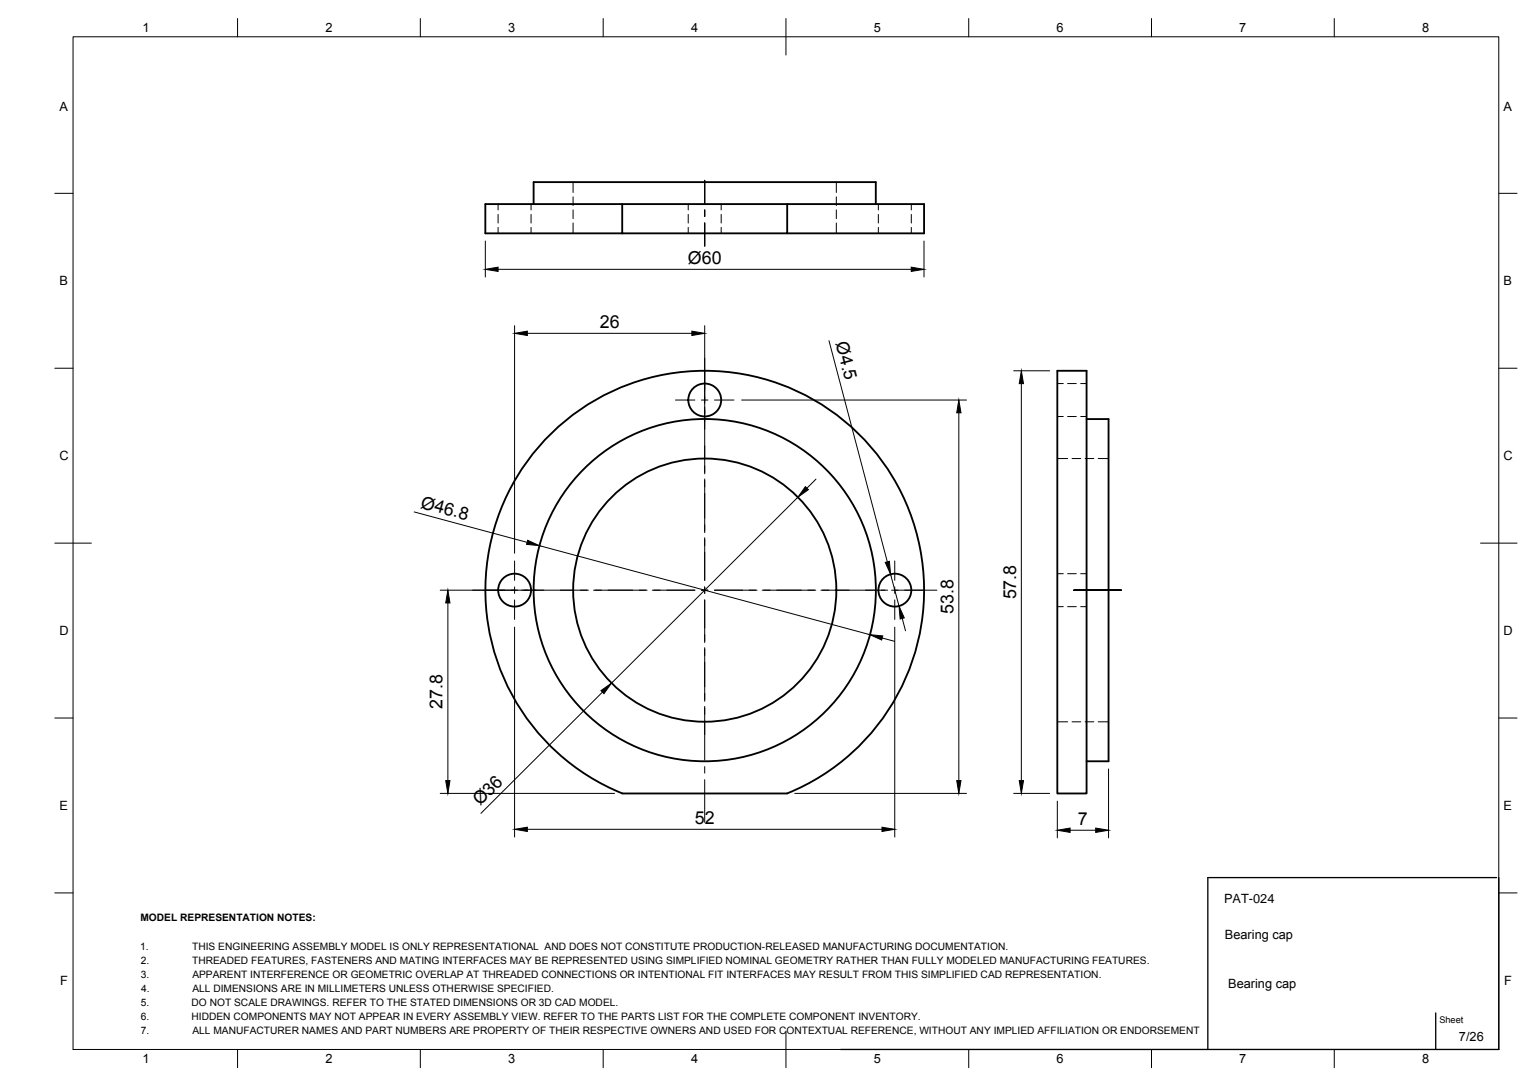
ISO-10303-21;
HEADER;
/* Generated by software containing ST-Developer
 * from STEP Tools, Inc. (www.steptools.com) 
 */

FILE_DESCRIPTION(
/* description */ ('Compact handwheel screw vise'),
/* implementation_level */ '2;1');

FILE_NAME(
/* name */ 'Bearing cap.step',
/* time_stamp */ '2026-10-29T16:08:22-07:00',
/* author */ (''),
/* organization */ (''),
/* preprocessor_version */ 'ST-DEVELOPER v20.2',
/* originating_system */ 'Autodesk Translation Framework v15.17.0.0',
/* authorisation */ '');

FILE_SCHEMA (('AUTOMOTIVE_DESIGN { 1 0 10303 214 3 1 1 }'));
ENDSEC;

DATA;
#10=MECHANICAL_DESIGN_GEOMETRIC_PRESENTATION_REPRESENTATION('',(#648),#25074);
#592=SHAPE_REPRESENTATION_RELATIONSHIP('SRR','None',#25200,#620);
#620=ADVANCED_BREP_SHAPE_REPRESENTATION('',(#684),#25047);
#648=STYLED_ITEM('',(#25439),#684);
#684=MANIFOLD_SOLID_BREP('Body1',#8056);
#744=FACE_BOUND('',#1574,.T.);
#745=FACE_BOUND('',#1575,.T.);
#746=FACE_BOUND('',#1576,.T.);
#747=FACE_BOUND('',#1577,.T.);
#748=FACE_BOUND('',#1581,.T.);
#749=FACE_BOUND('',#1584,.T.);
#750=FACE_BOUND('',#1585,.T.);
#751=FACE_BOUND('',#1586,.T.);
#752=FACE_BOUND('',#1587,.T.);
#856=PLANE('',#8514);
#857=PLANE('',#8515);
#858=PLANE('',#8522);
#859=PLANE('',#8526);
#1067=FACE_OUTER_BOUND('',#1569,.T.);
#1068=FACE_OUTER_BOUND('',#1570,.T.);
#1069=FACE_OUTER_BOUND('',#1571,.T.);
#1070=FACE_OUTER_BOUND('',#1572,.T.);
#1071=FACE_OUTER_BOUND('',#1573,.T.);
#1072=FACE_OUTER_BOUND('',#1578,.T.);
#1073=FACE_OUTER_BOUND('',#1579,.T.);
#1074=FACE_OUTER_BOUND('',#1580,.T.);
#1075=FACE_OUTER_BOUND('',#1582,.T.);
#1076=FACE_OUTER_BOUND('',#1583,.T.);
#1569=EDGE_LOOP('',(#5381,#5382,#5383,#5384));
#1570=EDGE_LOOP('',(#5385,#5386,#5387,#5388));
#1571=EDGE_LOOP('',(#5389,#5390,#5391,#5392));
#1572=EDGE_LOOP('',(#5393,#5394,#5395,#5396));
#1573=EDGE_LOOP('',(#5397,#5398));
#1574=EDGE_LOOP('',(#5399));
#1575=EDGE_LOOP('',(#5400));
#1576=EDGE_LOOP('',(#5401));
#1577=EDGE_LOOP('',(#5402));
#1578=EDGE_LOOP('',(#5403,#5404,#5405,#5406));
#1579=EDGE_LOOP('',(#5407,#5408,#5409,#5410));
#1580=EDGE_LOOP('',(#5411));
#1581=EDGE_LOOP('',(#5412));
#1582=EDGE_LOOP('',(#5413,#5414,#5415,#5416));
#1583=EDGE_LOOP('',(#5417,#5418));
#1584=EDGE_LOOP('',(#5419));
#1585=EDGE_LOOP('',(#5420));
#1586=EDGE_LOOP('',(#5421));
#1587=EDGE_LOOP('',(#5422));
#2131=LINE('',#11569,#2639);
#2132=LINE('',#11575,#2640);
#2133=LINE('',#11581,#2641);
#2134=LINE('',#11586,#2642);
#2135=LINE('',#11588,#2643);
#2136=LINE('',#11590,#2644);
#2137=LINE('',#11591,#2645);
#2138=LINE('',#11600,#2646);
#2139=LINE('',#11608,#2647);
#2639=VECTOR('',#9485,0.225);
#2640=VECTOR('',#9492,0.225);
#2641=VECTOR('',#9499,0.225);
#2642=VECTOR('',#9504,1.);
#2643=VECTOR('',#9505,1.);
#2644=VECTOR('',#9506,1.);
#2645=VECTOR('',#9507,1.);
#2646=VECTOR('',#9520,2.34);
#2647=VECTOR('',#9531,1.8);
#3120=CIRCLE('',#8506,0.225);
#3121=CIRCLE('',#8507,0.225);
#3122=CIRCLE('',#8509,0.225);
#3123=CIRCLE('',#8510,0.225);
#3124=CIRCLE('',#8512,0.225);
#3125=CIRCLE('',#8513,0.225);
#3126=CIRCLE('',#8516,3.);
#3127=CIRCLE('',#8517,2.34);
#3128=CIRCLE('',#8519,3.);
#3129=CIRCLE('',#8521,2.34);
#3130=CIRCLE('',#8523,1.8);
#3131=CIRCLE('',#8525,1.8);
#3407=VERTEX_POINT('',#11566);
#3408=VERTEX_POINT('',#11568);
#3409=VERTEX_POINT('',#11572);
#3410=VERTEX_POINT('',#11574);
#3411=VERTEX_POINT('',#11578);
#3412=VERTEX_POINT('',#11580);
#3413=VERTEX_POINT('',#11584);
#3414=VERTEX_POINT('',#11585);
#3415=VERTEX_POINT('',#11587);
#3416=VERTEX_POINT('',#11589);
#3417=VERTEX_POINT('',#11594);
#3418=VERTEX_POINT('',#11599);
#3419=VERTEX_POINT('',#11603);
#3420=VERTEX_POINT('',#11606);
#4177=EDGE_CURVE('',#3407,#3407,#3120,.T.);
#4178=EDGE_CURVE('',#3407,#3408,#2131,.T.);
#4179=EDGE_CURVE('',#3408,#3408,#3121,.T.);
#4180=EDGE_CURVE('',#3409,#3409,#3122,.T.);
#4181=EDGE_CURVE('',#3409,#3410,#2132,.T.);
#4182=EDGE_CURVE('',#3410,#3410,#3123,.T.);
#4183=EDGE_CURVE('',#3411,#3411,#3124,.T.);
#4184=EDGE_CURVE('',#3411,#3412,#2133,.T.);
#4185=EDGE_CURVE('',#3412,#3412,#3125,.T.);
#4186=EDGE_CURVE('',#3413,#3414,#2134,.T.);
#4187=EDGE_CURVE('',#3415,#3413,#2135,.T.);
#4188=EDGE_CURVE('',#3416,#3415,#2136,.T.);
#4189=EDGE_CURVE('',#3414,#3416,#2137,.T.);
#4190=EDGE_CURVE('',#3415,#3413,#3126,.T.);
#4191=EDGE_CURVE('',#3417,#3417,#3127,.T.);
#4192=EDGE_CURVE('',#3416,#3414,#3128,.T.);
#4193=EDGE_CURVE('',#3417,#3418,#2138,.T.);
#4194=EDGE_CURVE('',#3418,#3418,#3129,.T.);
#4195=EDGE_CURVE('',#3419,#3419,#3130,.T.);
#4196=EDGE_CURVE('',#3420,#3420,#3131,.T.);
#4197=EDGE_CURVE('',#3420,#3419,#2139,.T.);
#5381=ORIENTED_EDGE('',*,*,#4177,.F.);
#5382=ORIENTED_EDGE('',*,*,#4178,.T.);
#5383=ORIENTED_EDGE('',*,*,#4179,.F.);
#5384=ORIENTED_EDGE('',*,*,#4178,.F.);
#5385=ORIENTED_EDGE('',*,*,#4180,.F.);
#5386=ORIENTED_EDGE('',*,*,#4181,.T.);
#5387=ORIENTED_EDGE('',*,*,#4182,.F.);
#5388=ORIENTED_EDGE('',*,*,#4181,.F.);
#5389=ORIENTED_EDGE('',*,*,#4183,.F.);
#5390=ORIENTED_EDGE('',*,*,#4184,.T.);
#5391=ORIENTED_EDGE('',*,*,#4185,.F.);
#5392=ORIENTED_EDGE('',*,*,#4184,.F.);
#5393=ORIENTED_EDGE('',*,*,#4186,.F.);
#5394=ORIENTED_EDGE('',*,*,#4187,.F.);
#5395=ORIENTED_EDGE('',*,*,#4188,.F.);
#5396=ORIENTED_EDGE('',*,*,#4189,.F.);
#5397=ORIENTED_EDGE('',*,*,#4187,.T.);
#5398=ORIENTED_EDGE('',*,*,#4190,.F.);
#5399=ORIENTED_EDGE('',*,*,#4177,.T.);
#5400=ORIENTED_EDGE('',*,*,#4180,.T.);
#5401=ORIENTED_EDGE('',*,*,#4183,.T.);
#5402=ORIENTED_EDGE('',*,*,#4191,.T.);
#5403=ORIENTED_EDGE('',*,*,#4188,.T.);
#5404=ORIENTED_EDGE('',*,*,#4190,.T.);
#5405=ORIENTED_EDGE('',*,*,#4186,.T.);
#5406=ORIENTED_EDGE('',*,*,#4192,.F.);
#5407=ORIENTED_EDGE('',*,*,#4191,.F.);
#5408=ORIENTED_EDGE('',*,*,#4193,.T.);
#5409=ORIENTED_EDGE('',*,*,#4194,.T.);
#5410=ORIENTED_EDGE('',*,*,#4193,.F.);
#5411=ORIENTED_EDGE('',*,*,#4194,.F.);
#5412=ORIENTED_EDGE('',*,*,#4195,.F.);
#5413=ORIENTED_EDGE('',*,*,#4196,.F.);
#5414=ORIENTED_EDGE('',*,*,#4197,.T.);
#5415=ORIENTED_EDGE('',*,*,#4195,.T.);
#5416=ORIENTED_EDGE('',*,*,#4197,.F.);
#5417=ORIENTED_EDGE('',*,*,#4189,.T.);
#5418=ORIENTED_EDGE('',*,*,#4192,.T.);
#5419=ORIENTED_EDGE('',*,*,#4179,.T.);
#5420=ORIENTED_EDGE('',*,*,#4182,.T.);
#5421=ORIENTED_EDGE('',*,*,#4185,.T.);
#5422=ORIENTED_EDGE('',*,*,#4196,.T.);
#7366=CYLINDRICAL_SURFACE('',#8505,0.225);
#7367=CYLINDRICAL_SURFACE('',#8508,0.225);
#7368=CYLINDRICAL_SURFACE('',#8511,0.225);
#7369=CYLINDRICAL_SURFACE('',#8518,3.);
#7370=CYLINDRICAL_SURFACE('',#8520,2.34);
#7371=CYLINDRICAL_SURFACE('',#8524,1.8);
#7637=ADVANCED_FACE('',(#1067),#7366,.F.);
#7638=ADVANCED_FACE('',(#1068),#7367,.F.);
#7639=ADVANCED_FACE('',(#1069),#7368,.F.);
#7640=ADVANCED_FACE('',(#1070),#856,.F.);
#7641=ADVANCED_FACE('',(#1071,#744,#745,#746,#747),#857,.F.);
#7642=ADVANCED_FACE('',(#1072),#7369,.T.);
#7643=ADVANCED_FACE('',(#1073),#7370,.T.);
#7644=ADVANCED_FACE('',(#1074,#748),#858,.F.);
#7645=ADVANCED_FACE('',(#1075),#7371,.F.);
#7646=ADVANCED_FACE('',(#1076,#749,#750,#751,#752),#859,.T.);
#8056=CLOSED_SHELL('',(#7637,#7638,#7639,#7640,#7641,#7642,#7643,#7644,
#7645,#7646));
#8504=AXIS2_PLACEMENT_3D('',#11564,#9479,#9480);
#8505=AXIS2_PLACEMENT_3D('',#11565,#9481,#9482);
#8506=AXIS2_PLACEMENT_3D('',#11567,#9483,#9484);
#8507=AXIS2_PLACEMENT_3D('',#11570,#9486,#9487);
#8508=AXIS2_PLACEMENT_3D('',#11571,#9488,#9489);
#8509=AXIS2_PLACEMENT_3D('',#11573,#9490,#9491);
#8510=AXIS2_PLACEMENT_3D('',#11576,#9493,#9494);
#8511=AXIS2_PLACEMENT_3D('',#11577,#9495,#9496);
#8512=AXIS2_PLACEMENT_3D('',#11579,#9497,#9498);
#8513=AXIS2_PLACEMENT_3D('',#11582,#9500,#9501);
#8514=AXIS2_PLACEMENT_3D('',#11583,#9502,#9503);
#8515=AXIS2_PLACEMENT_3D('',#11592,#9508,#9509);
#8516=AXIS2_PLACEMENT_3D('',#11593,#9510,#9511);
#8517=AXIS2_PLACEMENT_3D('',#11595,#9512,#9513);
#8518=AXIS2_PLACEMENT_3D('',#11596,#9514,#9515);
#8519=AXIS2_PLACEMENT_3D('',#11597,#9516,#9517);
#8520=AXIS2_PLACEMENT_3D('',#11598,#9518,#9519);
#8521=AXIS2_PLACEMENT_3D('',#11601,#9521,#9522);
#8522=AXIS2_PLACEMENT_3D('',#11602,#9523,#9524);
#8523=AXIS2_PLACEMENT_3D('',#11604,#9525,#9526);
#8524=AXIS2_PLACEMENT_3D('',#11605,#9527,#9528);
#8525=AXIS2_PLACEMENT_3D('',#11607,#9529,#9530);
#8526=AXIS2_PLACEMENT_3D('',#11609,#9532,#9533);
#9479=DIRECTION('axis',(0.,0.,1.));
#9480=DIRECTION('refdir',(1.,0.,0.));
#9481=DIRECTION('center_axis',(1.,0.,0.));
#9482=DIRECTION('ref_axis',(0.,0.,-1.));
#9483=DIRECTION('center_axis',(1.,0.,0.));
#9484=DIRECTION('ref_axis',(0.,0.,-1.));
#9485=DIRECTION('',(1.,0.,0.));
#9486=DIRECTION('center_axis',(-1.,0.,0.));
#9487=DIRECTION('ref_axis',(0.,0.,-1.));
#9488=DIRECTION('center_axis',(1.,0.,0.));
#9489=DIRECTION('ref_axis',(0.,0.,-1.));
#9490=DIRECTION('center_axis',(1.,0.,0.));
#9491=DIRECTION('ref_axis',(0.,0.,-1.));
#9492=DIRECTION('',(1.,0.,0.));
#9493=DIRECTION('center_axis',(-1.,0.,0.));
#9494=DIRECTION('ref_axis',(0.,0.,-1.));
#9495=DIRECTION('center_axis',(1.,0.,0.));
#9496=DIRECTION('ref_axis',(0.,0.,-1.));
#9497=DIRECTION('center_axis',(1.,0.,0.));
#9498=DIRECTION('ref_axis',(0.,0.,-1.));
#9499=DIRECTION('',(1.,0.,0.));
#9500=DIRECTION('center_axis',(-1.,0.,0.));
#9501=DIRECTION('ref_axis',(0.,0.,-1.));
#9502=DIRECTION('center_axis',(0.,0.,1.));
#9503=DIRECTION('ref_axis',(0.,-1.,0.));
#9504=DIRECTION('',(1.,0.,0.));
#9505=DIRECTION('',(0.,-1.,0.));
#9506=DIRECTION('',(-1.,0.,0.));
#9507=DIRECTION('',(0.,1.,0.));
#9508=DIRECTION('center_axis',(1.,0.,0.));
#9509=DIRECTION('ref_axis',(0.,0.,-1.));
#9510=DIRECTION('center_axis',(1.,0.,0.));
#9511=DIRECTION('ref_axis',(0.,0.,-1.));
#9512=DIRECTION('center_axis',(1.,0.,0.));
#9513=DIRECTION('ref_axis',(0.,0.,-1.));
#9514=DIRECTION('center_axis',(1.,0.,0.));
#9515=DIRECTION('ref_axis',(0.,1.22464679914735E-16,1.));
#9516=DIRECTION('center_axis',(1.,0.,0.));
#9517=DIRECTION('ref_axis',(0.,0.,-1.));
#9518=DIRECTION('center_axis',(1.,0.,0.));
#9519=DIRECTION('ref_axis',(0.,0.,-1.));
#9520=DIRECTION('',(-1.,0.,0.));
#9521=DIRECTION('center_axis',(1.,0.,0.));
#9522=DIRECTION('ref_axis',(0.,0.,-1.));
#9523=DIRECTION('center_axis',(1.,0.,0.));
#9524=DIRECTION('ref_axis',(0.,0.,-1.));
#9525=DIRECTION('center_axis',(-1.,0.,0.));
#9526=DIRECTION('ref_axis',(0.,0.,-1.));
#9527=DIRECTION('center_axis',(1.,0.,0.));
#9528=DIRECTION('ref_axis',(0.,0.,-1.));
#9529=DIRECTION('center_axis',(-1.,0.,0.));
#9530=DIRECTION('ref_axis',(0.,0.,-1.));
#9531=DIRECTION('',(-1.,0.,0.));
#9532=DIRECTION('center_axis',(1.,0.,0.));
#9533=DIRECTION('ref_axis',(0.,0.,-1.));
#11564=CARTESIAN_POINT('',(0.,0.,0.));
#11565=CARTESIAN_POINT('Origin',(24.9,2.6,4.));
#11566=CARTESIAN_POINT('',(25.,2.6,4.225));
#11567=CARTESIAN_POINT('Origin',(25.,2.6,4.));
#11568=CARTESIAN_POINT('',(25.4,2.6,4.225));
#11569=CARTESIAN_POINT('',(24.9,2.6,4.225));
#11570=CARTESIAN_POINT('Origin',(25.4,2.6,4.));
#11571=CARTESIAN_POINT('Origin',(24.9,1.59204083889156E-16,6.6));
#11572=CARTESIAN_POINT('',(25.,1.31649530908341E-16,6.825));
#11573=CARTESIAN_POINT('Origin',(25.,1.59204083889156E-16,6.6));
#11574=CARTESIAN_POINT('',(25.4,1.86758636869971E-16,6.825));
#11575=CARTESIAN_POINT('',(24.9,1.31649530908341E-16,6.825));
#11576=CARTESIAN_POINT('Origin',(25.4,1.59204083889156E-16,6.6));
#11577=CARTESIAN_POINT('Origin',(24.9,-2.6,4.));
#11578=CARTESIAN_POINT('',(25.,-2.6,4.225));
#11579=CARTESIAN_POINT('Origin',(25.,-2.6,4.));
#11580=CARTESIAN_POINT('',(25.4,-2.6,4.225));
#11581=CARTESIAN_POINT('',(24.9,-2.6,4.225));
#11582=CARTESIAN_POINT('Origin',(25.4,-2.6,4.));
#11583=CARTESIAN_POINT('Origin',(24.9,3.5,1.22));
#11584=CARTESIAN_POINT('',(25.,-1.12765242872084,1.22));
#11585=CARTESIAN_POINT('',(25.4,-1.12765242872084,1.22));
#11586=CARTESIAN_POINT('',(25.,-1.12765242872084,1.22));
#11587=CARTESIAN_POINT('',(25.,1.12765242872084,1.22));
#11588=CARTESIAN_POINT('',(25.,1.75,1.22));
#11589=CARTESIAN_POINT('',(25.4,1.12765242872084,1.22));
#11590=CARTESIAN_POINT('',(25.,1.12765242872084,1.22));
#11591=CARTESIAN_POINT('',(25.4,1.75,1.22));
#11592=CARTESIAN_POINT('Origin',(25.,0.,4.));
#11593=CARTESIAN_POINT('Origin',(25.,0.,4.));
#11594=CARTESIAN_POINT('',(25.,-2.86567351000481E-16,6.34));
#11595=CARTESIAN_POINT('Origin',(25.,0.,4.));
#11596=CARTESIAN_POINT('Origin',(25.,0.,4.));
#11597=CARTESIAN_POINT('Origin',(25.4,0.,4.));
#11598=CARTESIAN_POINT('Origin',(24.7,0.,4.));
#11599=CARTESIAN_POINT('',(24.7,-2.86567351000481E-16,6.34));
#11600=CARTESIAN_POINT('',(24.7,-2.86567351000481E-16,6.34));
#11601=CARTESIAN_POINT('Origin',(24.7,0.,4.));
#11602=CARTESIAN_POINT('Origin',(24.7,0.,4.));
#11603=CARTESIAN_POINT('',(24.7,-2.20436423846524E-16,5.8));
#11604=CARTESIAN_POINT('Origin',(24.7,0.,4.));
#11605=CARTESIAN_POINT('Origin',(25.,0.,4.));
#11606=CARTESIAN_POINT('',(25.4,-2.20436423846524E-16,5.8));
#11607=CARTESIAN_POINT('Origin',(25.4,0.,4.));
#11608=CARTESIAN_POINT('',(25.,-2.20436423846524E-16,5.8));
#11609=CARTESIAN_POINT('Origin',(25.4,0.,4.));
#25013=UNCERTAINTY_MEASURE_WITH_UNIT(LENGTH_MEASURE(0.001),#25075,
'DISTANCE_ACCURACY_VALUE',
'Maximum model space distance between geometric entities at asserted c
onnectivities');
#25040=UNCERTAINTY_MEASURE_WITH_UNIT(LENGTH_MEASURE(0.001),#25075,
'DISTANCE_ACCURACY_VALUE',
'Maximum model space distance between geometric entities at asserted c
onnectivities');
#25047=(
GEOMETRIC_REPRESENTATION_CONTEXT(3)
GLOBAL_UNCERTAINTY_ASSIGNED_CONTEXT((#25013))
GLOBAL_UNIT_ASSIGNED_CONTEXT((#25075,#25077,#25078))
REPRESENTATION_CONTEXT('','3D')
);
#25074=(
GEOMETRIC_REPRESENTATION_CONTEXT(3)
GLOBAL_UNCERTAINTY_ASSIGNED_CONTEXT((#25040))
GLOBAL_UNIT_ASSIGNED_CONTEXT((#25075,#25077,#25078))
REPRESENTATION_CONTEXT('','3D')
);
#25075=(
LENGTH_UNIT()
NAMED_UNIT(*)
SI_UNIT(.CENTI.,.METRE.)
);
#25077=(
NAMED_UNIT(*)
PLANE_ANGLE_UNIT()
SI_UNIT($,.RADIAN.)
);
#25078=(
NAMED_UNIT(*)
SI_UNIT($,.STERADIAN.)
SOLID_ANGLE_UNIT()
);
#25085=SHAPE_DEFINITION_REPRESENTATION(#25118,#25200);
#25118=PRODUCT_DEFINITION_SHAPE('',$,#25234);
#25200=SHAPE_REPRESENTATION('',(#8504),#25047);
#25227=PRODUCT_DEFINITION_CONTEXT('part definition',#25328,'design');
#25234=PRODUCT_DEFINITION('Bearing cap','Bearing cap',#25267,#25227);
#25267=PRODUCT_DEFINITION_FORMATION('',$,#25336);
#25328=APPLICATION_CONTEXT(
'Core Data for Automotive Mechanical Design Process');
#25329=PRODUCT_CONTEXT('part definition',#25328,'mechanical');
#25336=PRODUCT('Bearing cap','Bearing cap','Bearing cap',(#25329));
#25433=COLOUR_RGB('Grey',0.48,0.52,0.57);
#25434=FILL_AREA_STYLE_COLOUR('',#25433);
#25435=FILL_AREA_STYLE('',(#25434));
#25436=SURFACE_STYLE_FILL_AREA(#25435);
#25437=SURFACE_SIDE_STYLE('',(#25436));
#25438=SURFACE_STYLE_USAGE(.BOTH.,#25437);
#25439=PRESENTATION_STYLE_ASSIGNMENT((#25438));
ENDSEC;
END-ISO-10303-21;
